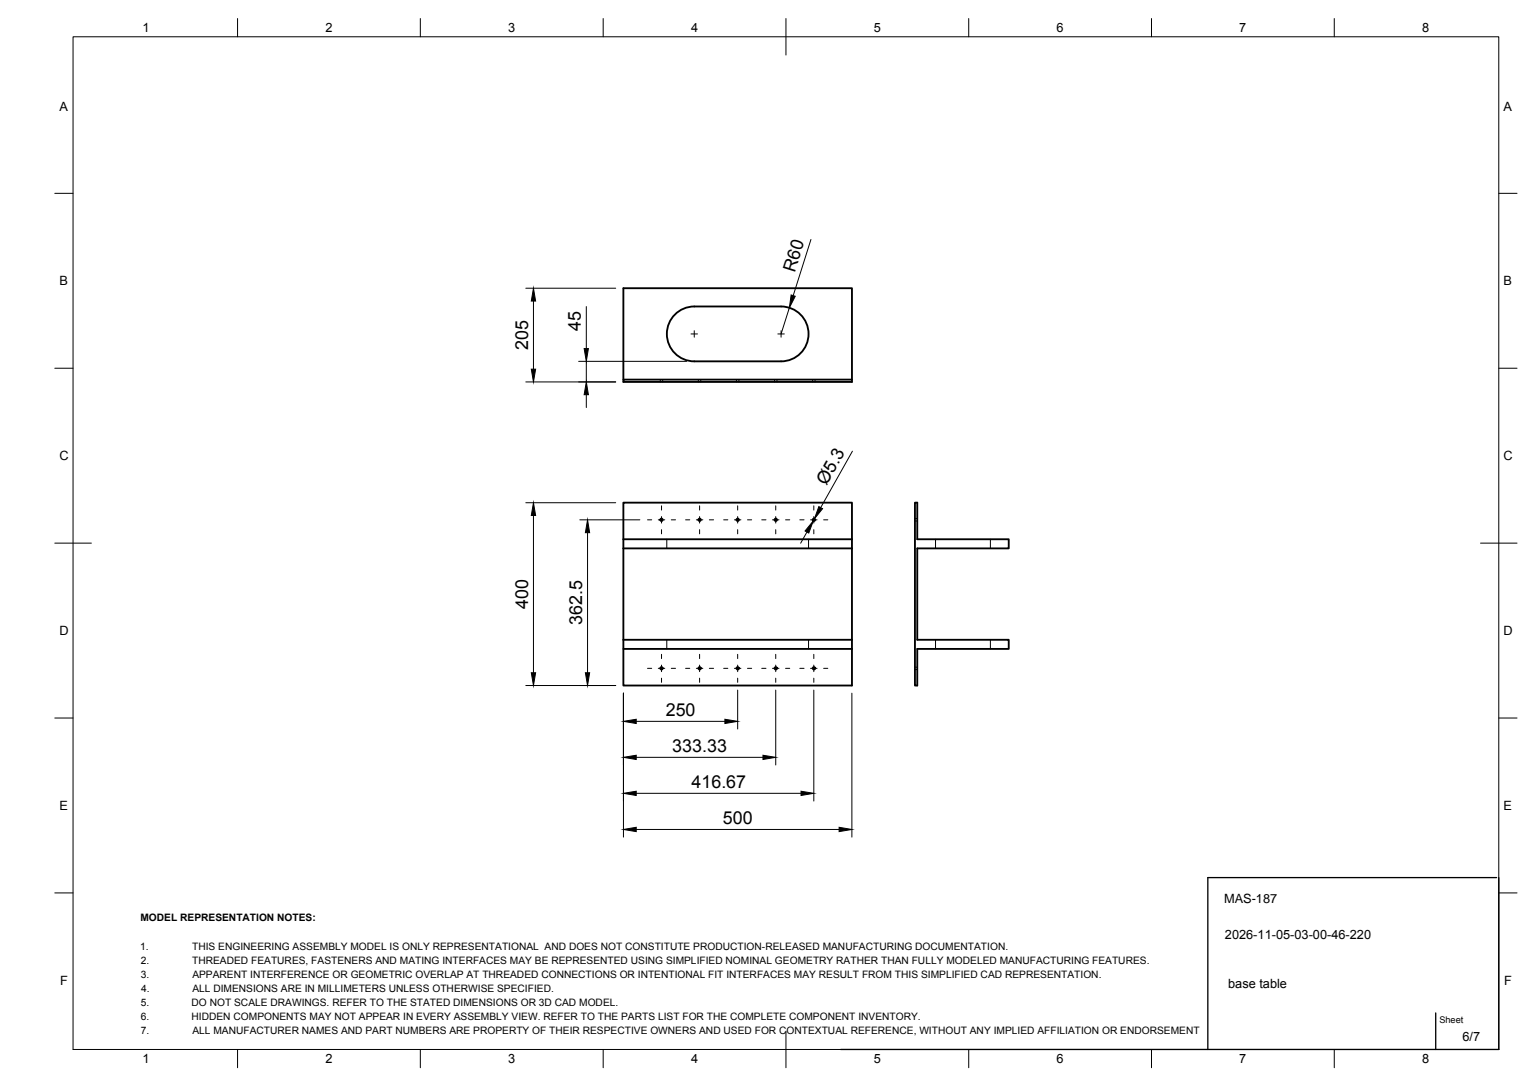
ISO-10303-21;
HEADER;
/* Generated by software containing ST-Developer
 * from STEP Tools, Inc. (www.steptools.com) 
 */

FILE_DESCRIPTION(
/* description */ ('STEP AP214'),
/* implementation_level */ '2;1');

FILE_NAME(
/* name */ 'base table.step',
/* time_stamp */ '2026-11-04T19:00:26-08:00',
/* author */ (''),
/* organization */ (''),
/* preprocessor_version */ 'ST-DEVELOPER v20.2',
/* originating_system */ 'Autodesk Translation Framework v15.17.0.0',
/* authorisation */ '');

FILE_SCHEMA (('AUTOMOTIVE_DESIGN { 1 0 10303 214 3 1 1 }'));
ENDSEC;

DATA;
#10=MECHANICAL_DESIGN_GEOMETRIC_PRESENTATION_REPRESENTATION('',(#271),#5689);
#257=SHAPE_REPRESENTATION_RELATIONSHIP('SRR','None',#5758,#264);
#264=ADVANCED_BREP_SHAPE_REPRESENTATION('',(#278),#5682);
#271=STYLED_ITEM('',(#5802),#278);
#278=MANIFOLD_SOLID_BREP('Body1',#2961);
#285=FACE_BOUND('',#615,.T.);
#286=FACE_BOUND('',#616,.T.);
#287=FACE_BOUND('',#617,.T.);
#288=FACE_BOUND('',#618,.T.);
#289=FACE_BOUND('',#619,.T.);
#290=FACE_BOUND('',#621,.T.);
#291=FACE_BOUND('',#622,.T.);
#292=FACE_BOUND('',#623,.T.);
#293=FACE_BOUND('',#624,.T.);
#294=FACE_BOUND('',#625,.T.);
#295=FACE_BOUND('',#628,.T.);
#296=FACE_BOUND('',#629,.T.);
#297=FACE_BOUND('',#630,.T.);
#298=FACE_BOUND('',#631,.T.);
#299=FACE_BOUND('',#632,.T.);
#300=FACE_BOUND('',#633,.T.);
#301=FACE_BOUND('',#634,.T.);
#302=FACE_BOUND('',#635,.T.);
#303=FACE_BOUND('',#636,.T.);
#304=FACE_BOUND('',#637,.T.);
#305=FACE_BOUND('',#642,.T.);
#306=FACE_BOUND('',#644,.T.);
#307=FACE_BOUND('',#647,.T.);
#308=FACE_BOUND('',#649,.T.);
#343=PLANE('',#3084);
#344=PLANE('',#3085);
#345=PLANE('',#3086);
#346=PLANE('',#3087);
#347=PLANE('',#3088);
#348=PLANE('',#3089);
#349=PLANE('',#3090);
#350=PLANE('',#3091);
#351=PLANE('',#3092);
#352=PLANE('',#3094);
#353=PLANE('',#3096);
#354=PLANE('',#3097);
#355=PLANE('',#3099);
#356=PLANE('',#3101);
#357=PLANE('',#3102);
#358=PLANE('',#3103);
#359=PLANE('',#3106);
#360=PLANE('',#3107);
#442=FACE_OUTER_BOUND('',#601,.T.);
#443=FACE_OUTER_BOUND('',#602,.T.);
#444=FACE_OUTER_BOUND('',#603,.T.);
#445=FACE_OUTER_BOUND('',#604,.T.);
#446=FACE_OUTER_BOUND('',#605,.T.);
#447=FACE_OUTER_BOUND('',#606,.T.);
#448=FACE_OUTER_BOUND('',#607,.T.);
#449=FACE_OUTER_BOUND('',#608,.T.);
#450=FACE_OUTER_BOUND('',#609,.T.);
#451=FACE_OUTER_BOUND('',#610,.T.);
#452=FACE_OUTER_BOUND('',#611,.T.);
#453=FACE_OUTER_BOUND('',#612,.T.);
#454=FACE_OUTER_BOUND('',#613,.T.);
#455=FACE_OUTER_BOUND('',#614,.T.);
#456=FACE_OUTER_BOUND('',#620,.T.);
#457=FACE_OUTER_BOUND('',#626,.T.);
#458=FACE_OUTER_BOUND('',#627,.T.);
#459=FACE_OUTER_BOUND('',#638,.T.);
#460=FACE_OUTER_BOUND('',#639,.T.);
#461=FACE_OUTER_BOUND('',#640,.T.);
#462=FACE_OUTER_BOUND('',#641,.T.);
#463=FACE_OUTER_BOUND('',#643,.T.);
#464=FACE_OUTER_BOUND('',#645,.T.);
#465=FACE_OUTER_BOUND('',#646,.T.);
#466=FACE_OUTER_BOUND('',#648,.T.);
#467=FACE_OUTER_BOUND('',#650,.T.);
#468=FACE_OUTER_BOUND('',#651,.T.);
#469=FACE_OUTER_BOUND('',#652,.T.);
#470=FACE_OUTER_BOUND('',#653,.T.);
#471=FACE_OUTER_BOUND('',#654,.T.);
#472=FACE_OUTER_BOUND('',#655,.T.);
#473=FACE_OUTER_BOUND('',#656,.T.);
#601=EDGE_LOOP('',(#2012,#2013,#2014,#2015));
#602=EDGE_LOOP('',(#2016,#2017,#2018,#2019));
#603=EDGE_LOOP('',(#2020,#2021,#2022,#2023));
#604=EDGE_LOOP('',(#2024,#2025,#2026,#2027));
#605=EDGE_LOOP('',(#2028,#2029,#2030,#2031));
#606=EDGE_LOOP('',(#2032,#2033,#2034,#2035));
#607=EDGE_LOOP('',(#2036,#2037,#2038,#2039));
#608=EDGE_LOOP('',(#2040,#2041,#2042,#2043));
#609=EDGE_LOOP('',(#2044,#2045,#2046,#2047));
#610=EDGE_LOOP('',(#2048,#2049,#2050,#2051));
#611=EDGE_LOOP('',(#2052,#2053,#2054,#2055));
#612=EDGE_LOOP('',(#2056,#2057,#2058,#2059));
#613=EDGE_LOOP('',(#2060,#2061,#2062,#2063));
#614=EDGE_LOOP('',(#2064,#2065,#2066,#2067));
#615=EDGE_LOOP('',(#2068));
#616=EDGE_LOOP('',(#2069));
#617=EDGE_LOOP('',(#2070));
#618=EDGE_LOOP('',(#2071));
#619=EDGE_LOOP('',(#2072));
#620=EDGE_LOOP('',(#2073,#2074,#2075,#2076));
#621=EDGE_LOOP('',(#2077));
#622=EDGE_LOOP('',(#2078));
#623=EDGE_LOOP('',(#2079));
#624=EDGE_LOOP('',(#2080));
#625=EDGE_LOOP('',(#2081));
#626=EDGE_LOOP('',(#2082,#2083,#2084,#2085,#2086,#2087,#2088,#2089,#2090,
#2091,#2092,#2093));
#627=EDGE_LOOP('',(#2094,#2095,#2096,#2097));
#628=EDGE_LOOP('',(#2098));
#629=EDGE_LOOP('',(#2099));
#630=EDGE_LOOP('',(#2100));
#631=EDGE_LOOP('',(#2101));
#632=EDGE_LOOP('',(#2102));
#633=EDGE_LOOP('',(#2103));
#634=EDGE_LOOP('',(#2104));
#635=EDGE_LOOP('',(#2105));
#636=EDGE_LOOP('',(#2106));
#637=EDGE_LOOP('',(#2107));
#638=EDGE_LOOP('',(#2108,#2109,#2110,#2111,#2112,#2113,#2114,#2115,#2116,
#2117,#2118,#2119));
#639=EDGE_LOOP('',(#2120,#2121,#2122,#2123));
#640=EDGE_LOOP('',(#2124,#2125,#2126,#2127));
#641=EDGE_LOOP('',(#2128,#2129,#2130,#2131));
#642=EDGE_LOOP('',(#2132,#2133,#2134,#2135));
#643=EDGE_LOOP('',(#2136,#2137,#2138,#2139));
#644=EDGE_LOOP('',(#2140,#2141,#2142,#2143));
#645=EDGE_LOOP('',(#2144,#2145,#2146,#2147));
#646=EDGE_LOOP('',(#2148,#2149,#2150,#2151));
#647=EDGE_LOOP('',(#2152,#2153,#2154,#2155));
#648=EDGE_LOOP('',(#2156,#2157,#2158,#2159));
#649=EDGE_LOOP('',(#2160,#2161,#2162,#2163));
#650=EDGE_LOOP('',(#2164,#2165,#2166,#2167));
#651=EDGE_LOOP('',(#2168,#2169,#2170,#2171));
#652=EDGE_LOOP('',(#2172,#2173,#2174,#2175));
#653=EDGE_LOOP('',(#2176,#2177,#2178,#2179));
#654=EDGE_LOOP('',(#2180,#2181,#2182,#2183));
#655=EDGE_LOOP('',(#2184,#2185,#2186,#2187));
#656=EDGE_LOOP('',(#2188,#2189,#2190,#2191));
#818=LINE('',#4253,#1049);
#819=LINE('',#4256,#1050);
#820=LINE('',#4262,#1051);
#821=LINE('',#4265,#1052);
#822=LINE('',#4270,#1053);
#823=LINE('',#4276,#1054);
#824=LINE('',#4282,#1055);
#825=LINE('',#4288,#1056);
#826=LINE('',#4294,#1057);
#827=LINE('',#4300,#1058);
#828=LINE('',#4306,#1059);
#829=LINE('',#4312,#1060);
#830=LINE('',#4318,#1061);
#831=LINE('',#4324,#1062);
#832=LINE('',#4329,#1063);
#833=LINE('',#4331,#1064);
#834=LINE('',#4333,#1065);
#835=LINE('',#4334,#1066);
#836=LINE('',#4338,#1067);
#837=LINE('',#4340,#1068);
#838=LINE('',#4342,#1069);
#839=LINE('',#4343,#1070);
#840=LINE('',#4347,#1071);
#841=LINE('',#4349,#1072);
#842=LINE('',#4351,#1073);
#843=LINE('',#4352,#1074);
#844=LINE('',#4355,#1075);
#845=LINE('',#4357,#1076);
#846=LINE('',#4358,#1077);
#847=LINE('',#4360,#1078);
#848=LINE('',#4362,#1079);
#849=LINE('',#4363,#1080);
#850=LINE('',#4365,#1081);
#851=LINE('',#4367,#1082);
#852=LINE('',#4368,#1083);
#853=LINE('',#4371,#1084);
#854=LINE('',#4373,#1085);
#855=LINE('',#4374,#1086);
#856=LINE('',#4376,#1087);
#857=LINE('',#4378,#1088);
#858=LINE('',#4380,#1089);
#859=LINE('',#4381,#1090);
#860=LINE('',#4383,#1091);
#861=LINE('',#4385,#1092);
#862=LINE('',#4386,#1093);
#863=LINE('',#4387,#1094);
#864=LINE('',#4391,#1095);
#865=LINE('',#4393,#1096);
#866=LINE('',#4396,#1097);
#867=LINE('',#4398,#1098);
#868=LINE('',#4402,#1099);
#869=LINE('',#4403,#1100);
#870=LINE('',#4406,#1101);
#871=LINE('',#4408,#1102);
#872=LINE('',#4411,#1103);
#873=LINE('',#4413,#1104);
#874=LINE('',#4417,#1105);
#875=LINE('',#4418,#1106);
#876=LINE('',#4421,#1107);
#877=LINE('',#4423,#1108);
#878=LINE('',#4426,#1109);
#879=LINE('',#4427,#1110);
#1049=VECTOR('',#3377,1000.);
#1050=VECTOR('',#3380,1000.);
#1051=VECTOR('',#3385,1000.);
#1052=VECTOR('',#3388,1000.);
#1053=VECTOR('',#3393,2.64999999999999);
#1054=VECTOR('',#3400,2.64999999999999);
#1055=VECTOR('',#3407,2.64999999999999);
#1056=VECTOR('',#3414,2.64999999999999);
#1057=VECTOR('',#3421,2.64999999999999);
#1058=VECTOR('',#3428,2.64999999999999);
#1059=VECTOR('',#3435,2.64999999999999);
#1060=VECTOR('',#3442,2.64999999999999);
#1061=VECTOR('',#3449,2.64999999999999);
#1062=VECTOR('',#3456,2.64999999999999);
#1063=VECTOR('',#3461,1000.);
#1064=VECTOR('',#3462,1000.);
#1065=VECTOR('',#3463,1000.);
#1066=VECTOR('',#3464,1000.);
#1067=VECTOR('',#3467,1000.);
#1068=VECTOR('',#3468,1000.);
#1069=VECTOR('',#3469,1000.);
#1070=VECTOR('',#3470,1000.);
#1071=VECTOR('',#3473,1000.);
#1072=VECTOR('',#3474,1000.);
#1073=VECTOR('',#3475,1000.);
#1074=VECTOR('',#3476,1000.);
#1075=VECTOR('',#3479,1000.);
#1076=VECTOR('',#3480,1000.);
#1077=VECTOR('',#3481,1000.);
#1078=VECTOR('',#3482,1000.);
#1079=VECTOR('',#3483,1000.);
#1080=VECTOR('',#3484,1000.);
#1081=VECTOR('',#3485,1000.);
#1082=VECTOR('',#3486,1000.);
#1083=VECTOR('',#3487,1000.);
#1084=VECTOR('',#3490,1000.);
#1085=VECTOR('',#3491,1000.);
#1086=VECTOR('',#3492,1000.);
#1087=VECTOR('',#3495,1000.);
#1088=VECTOR('',#3496,1000.);
#1089=VECTOR('',#3497,1000.);
#1090=VECTOR('',#3498,1000.);
#1091=VECTOR('',#3499,1000.);
#1092=VECTOR('',#3500,1000.);
#1093=VECTOR('',#3501,1000.);
#1094=VECTOR('',#3502,1000.);
#1095=VECTOR('',#3509,1000.);
#1096=VECTOR('',#3510,1000.);
#1097=VECTOR('',#3513,1000.);
#1098=VECTOR('',#3516,1000.);
#1099=VECTOR('',#3519,1000.);
#1100=VECTOR('',#3520,1000.);
#1101=VECTOR('',#3525,1000.);
#1102=VECTOR('',#3526,1000.);
#1103=VECTOR('',#3529,1000.);
#1104=VECTOR('',#3532,1000.);
#1105=VECTOR('',#3535,1000.);
#1106=VECTOR('',#3536,1000.);
#1107=VECTOR('',#3541,1000.);
#1108=VECTOR('',#3544,1000.);
#1109=VECTOR('',#3549,1000.);
#1110=VECTOR('',#3550,1000.);
#1280=CIRCLE('',#3049,60.);
#1281=CIRCLE('',#3050,60.);
#1282=CIRCLE('',#3052,60.);
#1283=CIRCLE('',#3053,60.);
#1284=CIRCLE('',#3055,2.64999999999999);
#1285=CIRCLE('',#3056,2.64999999999999);
#1286=CIRCLE('',#3058,2.64999999999999);
#1287=CIRCLE('',#3059,2.64999999999999);
#1288=CIRCLE('',#3061,2.64999999999999);
#1289=CIRCLE('',#3062,2.64999999999999);
#1290=CIRCLE('',#3064,2.64999999999999);
#1291=CIRCLE('',#3065,2.64999999999999);
#1292=CIRCLE('',#3067,2.64999999999999);
#1293=CIRCLE('',#3068,2.64999999999999);
#1294=CIRCLE('',#3070,2.64999999999999);
#1295=CIRCLE('',#3071,2.64999999999999);
#1296=CIRCLE('',#3073,2.64999999999999);
#1297=CIRCLE('',#3074,2.64999999999999);
#1298=CIRCLE('',#3076,2.64999999999999);
#1299=CIRCLE('',#3077,2.64999999999999);
#1300=CIRCLE('',#3079,2.64999999999999);
#1301=CIRCLE('',#3080,2.64999999999999);
#1302=CIRCLE('',#3082,2.64999999999999);
#1303=CIRCLE('',#3083,2.64999999999999);
#1304=CIRCLE('',#3093,60.);
#1305=CIRCLE('',#3095,60.);
#1306=CIRCLE('',#3098,60.);
#1307=CIRCLE('',#3100,60.);
#1395=VERTEX_POINT('',#4249);
#1396=VERTEX_POINT('',#4250);
#1397=VERTEX_POINT('',#4252);
#1398=VERTEX_POINT('',#4254);
#1399=VERTEX_POINT('',#4258);
#1400=VERTEX_POINT('',#4259);
#1401=VERTEX_POINT('',#4261);
#1402=VERTEX_POINT('',#4263);
#1403=VERTEX_POINT('',#4267);
#1404=VERTEX_POINT('',#4269);
#1405=VERTEX_POINT('',#4273);
#1406=VERTEX_POINT('',#4275);
#1407=VERTEX_POINT('',#4279);
#1408=VERTEX_POINT('',#4281);
#1409=VERTEX_POINT('',#4285);
#1410=VERTEX_POINT('',#4287);
#1411=VERTEX_POINT('',#4291);
#1412=VERTEX_POINT('',#4293);
#1413=VERTEX_POINT('',#4297);
#1414=VERTEX_POINT('',#4299);
#1415=VERTEX_POINT('',#4303);
#1416=VERTEX_POINT('',#4305);
#1417=VERTEX_POINT('',#4309);
#1418=VERTEX_POINT('',#4311);
#1419=VERTEX_POINT('',#4315);
#1420=VERTEX_POINT('',#4317);
#1421=VERTEX_POINT('',#4321);
#1422=VERTEX_POINT('',#4323);
#1423=VERTEX_POINT('',#4327);
#1424=VERTEX_POINT('',#4328);
#1425=VERTEX_POINT('',#4330);
#1426=VERTEX_POINT('',#4332);
#1427=VERTEX_POINT('',#4336);
#1428=VERTEX_POINT('',#4337);
#1429=VERTEX_POINT('',#4339);
#1430=VERTEX_POINT('',#4341);
#1431=VERTEX_POINT('',#4345);
#1432=VERTEX_POINT('',#4346);
#1433=VERTEX_POINT('',#4348);
#1434=VERTEX_POINT('',#4350);
#1435=VERTEX_POINT('',#4354);
#1436=VERTEX_POINT('',#4356);
#1437=VERTEX_POINT('',#4359);
#1438=VERTEX_POINT('',#4361);
#1439=VERTEX_POINT('',#4364);
#1440=VERTEX_POINT('',#4366);
#1441=VERTEX_POINT('',#4370);
#1442=VERTEX_POINT('',#4372);
#1443=VERTEX_POINT('',#4377);
#1444=VERTEX_POINT('',#4379);
#1445=VERTEX_POINT('',#4382);
#1446=VERTEX_POINT('',#4384);
#1447=VERTEX_POINT('',#4392);
#1448=VERTEX_POINT('',#4394);
#1449=VERTEX_POINT('',#4399);
#1450=VERTEX_POINT('',#4400);
#1451=VERTEX_POINT('',#4407);
#1452=VERTEX_POINT('',#4409);
#1453=VERTEX_POINT('',#4414);
#1454=VERTEX_POINT('',#4415);
#1634=EDGE_CURVE('',#1395,#1396,#1280,.T.);
#1635=EDGE_CURVE('',#1395,#1397,#818,.T.);
#1636=EDGE_CURVE('',#1397,#1398,#1281,.T.);
#1637=EDGE_CURVE('',#1396,#1398,#819,.T.);
#1638=EDGE_CURVE('',#1399,#1400,#1282,.T.);
#1639=EDGE_CURVE('',#1399,#1401,#820,.T.);
#1640=EDGE_CURVE('',#1401,#1402,#1283,.T.);
#1641=EDGE_CURVE('',#1400,#1402,#821,.T.);
#1642=EDGE_CURVE('',#1403,#1403,#1284,.T.);
#1643=EDGE_CURVE('',#1403,#1404,#822,.T.);
#1644=EDGE_CURVE('',#1404,#1404,#1285,.T.);
#1645=EDGE_CURVE('',#1405,#1405,#1286,.T.);
#1646=EDGE_CURVE('',#1405,#1406,#823,.T.);
#1647=EDGE_CURVE('',#1406,#1406,#1287,.T.);
#1648=EDGE_CURVE('',#1407,#1407,#1288,.T.);
#1649=EDGE_CURVE('',#1407,#1408,#824,.T.);
#1650=EDGE_CURVE('',#1408,#1408,#1289,.T.);
#1651=EDGE_CURVE('',#1409,#1409,#1290,.T.);
#1652=EDGE_CURVE('',#1409,#1410,#825,.T.);
#1653=EDGE_CURVE('',#1410,#1410,#1291,.T.);
#1654=EDGE_CURVE('',#1411,#1411,#1292,.T.);
#1655=EDGE_CURVE('',#1411,#1412,#826,.T.);
#1656=EDGE_CURVE('',#1412,#1412,#1293,.T.);
#1657=EDGE_CURVE('',#1413,#1413,#1294,.T.);
#1658=EDGE_CURVE('',#1413,#1414,#827,.T.);
#1659=EDGE_CURVE('',#1414,#1414,#1295,.T.);
#1660=EDGE_CURVE('',#1415,#1415,#1296,.T.);
#1661=EDGE_CURVE('',#1415,#1416,#828,.T.);
#1662=EDGE_CURVE('',#1416,#1416,#1297,.T.);
#1663=EDGE_CURVE('',#1417,#1417,#1298,.T.);
#1664=EDGE_CURVE('',#1417,#1418,#829,.T.);
#1665=EDGE_CURVE('',#1418,#1418,#1299,.T.);
#1666=EDGE_CURVE('',#1419,#1419,#1300,.T.);
#1667=EDGE_CURVE('',#1419,#1420,#830,.T.);
#1668=EDGE_CURVE('',#1420,#1420,#1301,.T.);
#1669=EDGE_CURVE('',#1421,#1421,#1302,.T.);
#1670=EDGE_CURVE('',#1421,#1422,#831,.T.);
#1671=EDGE_CURVE('',#1422,#1422,#1303,.T.);
#1672=EDGE_CURVE('',#1423,#1424,#832,.T.);
#1673=EDGE_CURVE('',#1423,#1425,#833,.T.);
#1674=EDGE_CURVE('',#1425,#1426,#834,.T.);
#1675=EDGE_CURVE('',#1424,#1426,#835,.T.);
#1676=EDGE_CURVE('',#1427,#1428,#836,.T.);
#1677=EDGE_CURVE('',#1427,#1429,#837,.T.);
#1678=EDGE_CURVE('',#1429,#1430,#838,.T.);
#1679=EDGE_CURVE('',#1428,#1430,#839,.T.);
#1680=EDGE_CURVE('',#1431,#1432,#840,.T.);
#1681=EDGE_CURVE('',#1432,#1433,#841,.T.);
#1682=EDGE_CURVE('',#1434,#1433,#842,.T.);
#1683=EDGE_CURVE('',#1431,#1434,#843,.T.);
#1684=EDGE_CURVE('',#1435,#1430,#844,.T.);
#1685=EDGE_CURVE('',#1436,#1435,#845,.T.);
#1686=EDGE_CURVE('',#1436,#1434,#846,.T.);
#1687=EDGE_CURVE('',#1437,#1433,#847,.T.);
#1688=EDGE_CURVE('',#1437,#1438,#848,.T.);
#1689=EDGE_CURVE('',#1438,#1424,#849,.T.);
#1690=EDGE_CURVE('',#1439,#1426,#850,.T.);
#1691=EDGE_CURVE('',#1439,#1440,#851,.T.);
#1692=EDGE_CURVE('',#1440,#1428,#852,.T.);
#1693=EDGE_CURVE('',#1441,#1435,#853,.T.);
#1694=EDGE_CURVE('',#1442,#1441,#854,.T.);
#1695=EDGE_CURVE('',#1442,#1436,#855,.T.);
#1696=EDGE_CURVE('',#1429,#1441,#856,.T.);
#1697=EDGE_CURVE('',#1443,#1427,#857,.T.);
#1698=EDGE_CURVE('',#1443,#1444,#858,.T.);
#1699=EDGE_CURVE('',#1444,#1425,#859,.T.);
#1700=EDGE_CURVE('',#1445,#1423,#860,.T.);
#1701=EDGE_CURVE('',#1445,#1446,#861,.T.);
#1702=EDGE_CURVE('',#1446,#1432,#862,.T.);
#1703=EDGE_CURVE('',#1431,#1442,#863,.T.);
#1704=EDGE_CURVE('',#1443,#1440,#864,.T.);
#1705=EDGE_CURVE('',#1396,#1447,#865,.T.);
#1706=EDGE_CURVE('',#1447,#1448,#1304,.T.);
#1707=EDGE_CURVE('',#1448,#1395,#866,.T.);
#1708=EDGE_CURVE('',#1444,#1439,#867,.T.);
#1709=EDGE_CURVE('',#1449,#1450,#1305,.T.);
#1710=EDGE_CURVE('',#1398,#1449,#868,.T.);
#1711=EDGE_CURVE('',#1450,#1397,#869,.T.);
#1712=EDGE_CURVE('',#1445,#1438,#870,.T.);
#1713=EDGE_CURVE('',#1400,#1451,#871,.T.);
#1714=EDGE_CURVE('',#1451,#1452,#1306,.T.);
#1715=EDGE_CURVE('',#1452,#1399,#872,.T.);
#1716=EDGE_CURVE('',#1446,#1437,#873,.T.);
#1717=EDGE_CURVE('',#1453,#1454,#1307,.T.);
#1718=EDGE_CURVE('',#1402,#1453,#874,.T.);
#1719=EDGE_CURVE('',#1454,#1401,#875,.T.);
#1720=EDGE_CURVE('',#1452,#1454,#876,.T.);
#1721=EDGE_CURVE('',#1451,#1453,#877,.T.);
#1722=EDGE_CURVE('',#1447,#1449,#878,.T.);
#1723=EDGE_CURVE('',#1448,#1450,#879,.T.);
#2012=ORIENTED_EDGE('',*,*,#1634,.F.);
#2013=ORIENTED_EDGE('',*,*,#1635,.T.);
#2014=ORIENTED_EDGE('',*,*,#1636,.T.);
#2015=ORIENTED_EDGE('',*,*,#1637,.F.);
#2016=ORIENTED_EDGE('',*,*,#1638,.F.);
#2017=ORIENTED_EDGE('',*,*,#1639,.T.);
#2018=ORIENTED_EDGE('',*,*,#1640,.T.);
#2019=ORIENTED_EDGE('',*,*,#1641,.F.);
#2020=ORIENTED_EDGE('',*,*,#1642,.T.);
#2021=ORIENTED_EDGE('',*,*,#1643,.T.);
#2022=ORIENTED_EDGE('',*,*,#1644,.F.);
#2023=ORIENTED_EDGE('',*,*,#1643,.F.);
#2024=ORIENTED_EDGE('',*,*,#1645,.T.);
#2025=ORIENTED_EDGE('',*,*,#1646,.T.);
#2026=ORIENTED_EDGE('',*,*,#1647,.F.);
#2027=ORIENTED_EDGE('',*,*,#1646,.F.);
#2028=ORIENTED_EDGE('',*,*,#1648,.T.);
#2029=ORIENTED_EDGE('',*,*,#1649,.T.);
#2030=ORIENTED_EDGE('',*,*,#1650,.F.);
#2031=ORIENTED_EDGE('',*,*,#1649,.F.);
#2032=ORIENTED_EDGE('',*,*,#1651,.T.);
#2033=ORIENTED_EDGE('',*,*,#1652,.T.);
#2034=ORIENTED_EDGE('',*,*,#1653,.F.);
#2035=ORIENTED_EDGE('',*,*,#1652,.F.);
#2036=ORIENTED_EDGE('',*,*,#1654,.T.);
#2037=ORIENTED_EDGE('',*,*,#1655,.T.);
#2038=ORIENTED_EDGE('',*,*,#1656,.F.);
#2039=ORIENTED_EDGE('',*,*,#1655,.F.);
#2040=ORIENTED_EDGE('',*,*,#1657,.F.);
#2041=ORIENTED_EDGE('',*,*,#1658,.T.);
#2042=ORIENTED_EDGE('',*,*,#1659,.T.);
#2043=ORIENTED_EDGE('',*,*,#1658,.F.);
#2044=ORIENTED_EDGE('',*,*,#1660,.F.);
#2045=ORIENTED_EDGE('',*,*,#1661,.T.);
#2046=ORIENTED_EDGE('',*,*,#1662,.T.);
#2047=ORIENTED_EDGE('',*,*,#1661,.F.);
#2048=ORIENTED_EDGE('',*,*,#1663,.F.);
#2049=ORIENTED_EDGE('',*,*,#1664,.T.);
#2050=ORIENTED_EDGE('',*,*,#1665,.T.);
#2051=ORIENTED_EDGE('',*,*,#1664,.F.);
#2052=ORIENTED_EDGE('',*,*,#1666,.F.);
#2053=ORIENTED_EDGE('',*,*,#1667,.T.);
#2054=ORIENTED_EDGE('',*,*,#1668,.T.);
#2055=ORIENTED_EDGE('',*,*,#1667,.F.);
#2056=ORIENTED_EDGE('',*,*,#1669,.F.);
#2057=ORIENTED_EDGE('',*,*,#1670,.T.);
#2058=ORIENTED_EDGE('',*,*,#1671,.T.);
#2059=ORIENTED_EDGE('',*,*,#1670,.F.);
#2060=ORIENTED_EDGE('',*,*,#1672,.F.);
#2061=ORIENTED_EDGE('',*,*,#1673,.T.);
#2062=ORIENTED_EDGE('',*,*,#1674,.T.);
#2063=ORIENTED_EDGE('',*,*,#1675,.F.);
#2064=ORIENTED_EDGE('',*,*,#1676,.F.);
#2065=ORIENTED_EDGE('',*,*,#1677,.T.);
#2066=ORIENTED_EDGE('',*,*,#1678,.T.);
#2067=ORIENTED_EDGE('',*,*,#1679,.F.);
#2068=ORIENTED_EDGE('',*,*,#1642,.F.);
#2069=ORIENTED_EDGE('',*,*,#1645,.F.);
#2070=ORIENTED_EDGE('',*,*,#1648,.F.);
#2071=ORIENTED_EDGE('',*,*,#1651,.F.);
#2072=ORIENTED_EDGE('',*,*,#1654,.F.);
#2073=ORIENTED_EDGE('',*,*,#1680,.T.);
#2074=ORIENTED_EDGE('',*,*,#1681,.T.);
#2075=ORIENTED_EDGE('',*,*,#1682,.F.);
#2076=ORIENTED_EDGE('',*,*,#1683,.F.);
#2077=ORIENTED_EDGE('',*,*,#1657,.T.);
#2078=ORIENTED_EDGE('',*,*,#1660,.T.);
#2079=ORIENTED_EDGE('',*,*,#1663,.T.);
#2080=ORIENTED_EDGE('',*,*,#1666,.T.);
#2081=ORIENTED_EDGE('',*,*,#1669,.T.);
#2082=ORIENTED_EDGE('',*,*,#1684,.F.);
#2083=ORIENTED_EDGE('',*,*,#1685,.F.);
#2084=ORIENTED_EDGE('',*,*,#1686,.T.);
#2085=ORIENTED_EDGE('',*,*,#1682,.T.);
#2086=ORIENTED_EDGE('',*,*,#1687,.F.);
#2087=ORIENTED_EDGE('',*,*,#1688,.T.);
#2088=ORIENTED_EDGE('',*,*,#1689,.T.);
#2089=ORIENTED_EDGE('',*,*,#1675,.T.);
#2090=ORIENTED_EDGE('',*,*,#1690,.F.);
#2091=ORIENTED_EDGE('',*,*,#1691,.T.);
#2092=ORIENTED_EDGE('',*,*,#1692,.T.);
#2093=ORIENTED_EDGE('',*,*,#1679,.T.);
#2094=ORIENTED_EDGE('',*,*,#1693,.F.);
#2095=ORIENTED_EDGE('',*,*,#1694,.F.);
#2096=ORIENTED_EDGE('',*,*,#1695,.T.);
#2097=ORIENTED_EDGE('',*,*,#1685,.T.);
#2098=ORIENTED_EDGE('',*,*,#1644,.T.);
#2099=ORIENTED_EDGE('',*,*,#1647,.T.);
#2100=ORIENTED_EDGE('',*,*,#1650,.T.);
#2101=ORIENTED_EDGE('',*,*,#1653,.T.);
#2102=ORIENTED_EDGE('',*,*,#1656,.T.);
#2103=ORIENTED_EDGE('',*,*,#1659,.F.);
#2104=ORIENTED_EDGE('',*,*,#1662,.F.);
#2105=ORIENTED_EDGE('',*,*,#1665,.F.);
#2106=ORIENTED_EDGE('',*,*,#1668,.F.);
#2107=ORIENTED_EDGE('',*,*,#1671,.F.);
#2108=ORIENTED_EDGE('',*,*,#1696,.F.);
#2109=ORIENTED_EDGE('',*,*,#1677,.F.);
#2110=ORIENTED_EDGE('',*,*,#1697,.F.);
#2111=ORIENTED_EDGE('',*,*,#1698,.T.);
#2112=ORIENTED_EDGE('',*,*,#1699,.T.);
#2113=ORIENTED_EDGE('',*,*,#1673,.F.);
#2114=ORIENTED_EDGE('',*,*,#1700,.F.);
#2115=ORIENTED_EDGE('',*,*,#1701,.T.);
#2116=ORIENTED_EDGE('',*,*,#1702,.T.);
#2117=ORIENTED_EDGE('',*,*,#1680,.F.);
#2118=ORIENTED_EDGE('',*,*,#1703,.T.);
#2119=ORIENTED_EDGE('',*,*,#1694,.T.);
#2120=ORIENTED_EDGE('',*,*,#1683,.T.);
#2121=ORIENTED_EDGE('',*,*,#1686,.F.);
#2122=ORIENTED_EDGE('',*,*,#1695,.F.);
#2123=ORIENTED_EDGE('',*,*,#1703,.F.);
#2124=ORIENTED_EDGE('',*,*,#1678,.F.);
#2125=ORIENTED_EDGE('',*,*,#1696,.T.);
#2126=ORIENTED_EDGE('',*,*,#1693,.T.);
#2127=ORIENTED_EDGE('',*,*,#1684,.T.);
#2128=ORIENTED_EDGE('',*,*,#1676,.T.);
#2129=ORIENTED_EDGE('',*,*,#1692,.F.);
#2130=ORIENTED_EDGE('',*,*,#1704,.F.);
#2131=ORIENTED_EDGE('',*,*,#1697,.T.);
#2132=ORIENTED_EDGE('',*,*,#1705,.T.);
#2133=ORIENTED_EDGE('',*,*,#1706,.T.);
#2134=ORIENTED_EDGE('',*,*,#1707,.T.);
#2135=ORIENTED_EDGE('',*,*,#1634,.T.);
#2136=ORIENTED_EDGE('',*,*,#1674,.F.);
#2137=ORIENTED_EDGE('',*,*,#1699,.F.);
#2138=ORIENTED_EDGE('',*,*,#1708,.T.);
#2139=ORIENTED_EDGE('',*,*,#1690,.T.);
#2140=ORIENTED_EDGE('',*,*,#1709,.F.);
#2141=ORIENTED_EDGE('',*,*,#1710,.F.);
#2142=ORIENTED_EDGE('',*,*,#1636,.F.);
#2143=ORIENTED_EDGE('',*,*,#1711,.F.);
#2144=ORIENTED_EDGE('',*,*,#1704,.T.);
#2145=ORIENTED_EDGE('',*,*,#1691,.F.);
#2146=ORIENTED_EDGE('',*,*,#1708,.F.);
#2147=ORIENTED_EDGE('',*,*,#1698,.F.);
#2148=ORIENTED_EDGE('',*,*,#1672,.T.);
#2149=ORIENTED_EDGE('',*,*,#1689,.F.);
#2150=ORIENTED_EDGE('',*,*,#1712,.F.);
#2151=ORIENTED_EDGE('',*,*,#1700,.T.);
#2152=ORIENTED_EDGE('',*,*,#1713,.T.);
#2153=ORIENTED_EDGE('',*,*,#1714,.T.);
#2154=ORIENTED_EDGE('',*,*,#1715,.T.);
#2155=ORIENTED_EDGE('',*,*,#1638,.T.);
#2156=ORIENTED_EDGE('',*,*,#1681,.F.);
#2157=ORIENTED_EDGE('',*,*,#1702,.F.);
#2158=ORIENTED_EDGE('',*,*,#1716,.T.);
#2159=ORIENTED_EDGE('',*,*,#1687,.T.);
#2160=ORIENTED_EDGE('',*,*,#1717,.F.);
#2161=ORIENTED_EDGE('',*,*,#1718,.F.);
#2162=ORIENTED_EDGE('',*,*,#1640,.F.);
#2163=ORIENTED_EDGE('',*,*,#1719,.F.);
#2164=ORIENTED_EDGE('',*,*,#1712,.T.);
#2165=ORIENTED_EDGE('',*,*,#1688,.F.);
#2166=ORIENTED_EDGE('',*,*,#1716,.F.);
#2167=ORIENTED_EDGE('',*,*,#1701,.F.);
#2168=ORIENTED_EDGE('',*,*,#1720,.T.);
#2169=ORIENTED_EDGE('',*,*,#1719,.T.);
#2170=ORIENTED_EDGE('',*,*,#1639,.F.);
#2171=ORIENTED_EDGE('',*,*,#1715,.F.);
#2172=ORIENTED_EDGE('',*,*,#1641,.T.);
#2173=ORIENTED_EDGE('',*,*,#1718,.T.);
#2174=ORIENTED_EDGE('',*,*,#1721,.F.);
#2175=ORIENTED_EDGE('',*,*,#1713,.F.);
#2176=ORIENTED_EDGE('',*,*,#1721,.T.);
#2177=ORIENTED_EDGE('',*,*,#1717,.T.);
#2178=ORIENTED_EDGE('',*,*,#1720,.F.);
#2179=ORIENTED_EDGE('',*,*,#1714,.F.);
#2180=ORIENTED_EDGE('',*,*,#1722,.T.);
#2181=ORIENTED_EDGE('',*,*,#1709,.T.);
#2182=ORIENTED_EDGE('',*,*,#1723,.F.);
#2183=ORIENTED_EDGE('',*,*,#1706,.F.);
#2184=ORIENTED_EDGE('',*,*,#1637,.T.);
#2185=ORIENTED_EDGE('',*,*,#1710,.T.);
#2186=ORIENTED_EDGE('',*,*,#1722,.F.);
#2187=ORIENTED_EDGE('',*,*,#1705,.F.);
#2188=ORIENTED_EDGE('',*,*,#1723,.T.);
#2189=ORIENTED_EDGE('',*,*,#1711,.T.);
#2190=ORIENTED_EDGE('',*,*,#1635,.F.);
#2191=ORIENTED_EDGE('',*,*,#1707,.F.);
#2768=CYLINDRICAL_SURFACE('',#3048,60.);
#2769=CYLINDRICAL_SURFACE('',#3051,60.);
#2770=CYLINDRICAL_SURFACE('',#3054,2.64999999999999);
#2771=CYLINDRICAL_SURFACE('',#3057,2.64999999999999);
#2772=CYLINDRICAL_SURFACE('',#3060,2.64999999999999);
#2773=CYLINDRICAL_SURFACE('',#3063,2.64999999999999);
#2774=CYLINDRICAL_SURFACE('',#3066,2.64999999999999);
#2775=CYLINDRICAL_SURFACE('',#3069,2.64999999999999);
#2776=CYLINDRICAL_SURFACE('',#3072,2.64999999999999);
#2777=CYLINDRICAL_SURFACE('',#3075,2.64999999999999);
#2778=CYLINDRICAL_SURFACE('',#3078,2.64999999999999);
#2779=CYLINDRICAL_SURFACE('',#3081,2.64999999999999);
#2780=CYLINDRICAL_SURFACE('',#3104,60.);
#2781=CYLINDRICAL_SURFACE('',#3105,60.);
#2802=ADVANCED_FACE('',(#442),#2768,.F.);
#2803=ADVANCED_FACE('',(#443),#2769,.F.);
#2804=ADVANCED_FACE('',(#444),#2770,.F.);
#2805=ADVANCED_FACE('',(#445),#2771,.F.);
#2806=ADVANCED_FACE('',(#446),#2772,.F.);
#2807=ADVANCED_FACE('',(#447),#2773,.F.);
#2808=ADVANCED_FACE('',(#448),#2774,.F.);
#2809=ADVANCED_FACE('',(#449),#2775,.F.);
#2810=ADVANCED_FACE('',(#450),#2776,.F.);
#2811=ADVANCED_FACE('',(#451),#2777,.F.);
#2812=ADVANCED_FACE('',(#452),#2778,.F.);
#2813=ADVANCED_FACE('',(#453),#2779,.F.);
#2814=ADVANCED_FACE('',(#454),#343,.F.);
#2815=ADVANCED_FACE('',(#455,#285,#286,#287,#288,#289),#344,.F.);
#2816=ADVANCED_FACE('',(#456,#290,#291,#292,#293,#294),#345,.F.);
#2817=ADVANCED_FACE('',(#457),#346,.T.);
#2818=ADVANCED_FACE('',(#458,#295,#296,#297,#298,#299,#300,#301,#302,#303,
#304),#347,.T.);
#2819=ADVANCED_FACE('',(#459),#348,.T.);
#2820=ADVANCED_FACE('',(#460),#349,.F.);
#2821=ADVANCED_FACE('',(#461),#350,.T.);
#2822=ADVANCED_FACE('',(#462,#305),#351,.F.);
#2823=ADVANCED_FACE('',(#463,#306),#352,.T.);
#2824=ADVANCED_FACE('',(#464),#353,.F.);
#2825=ADVANCED_FACE('',(#465,#307),#354,.F.);
#2826=ADVANCED_FACE('',(#466,#308),#355,.T.);
#2827=ADVANCED_FACE('',(#467),#356,.F.);
#2828=ADVANCED_FACE('',(#468),#357,.F.);
#2829=ADVANCED_FACE('',(#469),#358,.F.);
#2830=ADVANCED_FACE('',(#470),#2780,.F.);
#2831=ADVANCED_FACE('',(#471),#2781,.F.);
#2832=ADVANCED_FACE('',(#472),#359,.F.);
#2833=ADVANCED_FACE('',(#473),#360,.F.);
#2961=CLOSED_SHELL('',(#2802,#2803,#2804,#2805,#2806,#2807,#2808,#2809,
#2810,#2811,#2812,#2813,#2814,#2815,#2816,#2817,#2818,#2819,#2820,#2821,
#2822,#2823,#2824,#2825,#2826,#2827,#2828,#2829,#2830,#2831,#2832,#2833));
#3047=AXIS2_PLACEMENT_3D('',#4247,#3371,#3372);
#3048=AXIS2_PLACEMENT_3D('',#4248,#3373,#3374);
#3049=AXIS2_PLACEMENT_3D('',#4251,#3375,#3376);
#3050=AXIS2_PLACEMENT_3D('',#4255,#3378,#3379);
#3051=AXIS2_PLACEMENT_3D('',#4257,#3381,#3382);
#3052=AXIS2_PLACEMENT_3D('',#4260,#3383,#3384);
#3053=AXIS2_PLACEMENT_3D('',#4264,#3386,#3387);
#3054=AXIS2_PLACEMENT_3D('',#4266,#3389,#3390);
#3055=AXIS2_PLACEMENT_3D('',#4268,#3391,#3392);
#3056=AXIS2_PLACEMENT_3D('',#4271,#3394,#3395);
#3057=AXIS2_PLACEMENT_3D('',#4272,#3396,#3397);
#3058=AXIS2_PLACEMENT_3D('',#4274,#3398,#3399);
#3059=AXIS2_PLACEMENT_3D('',#4277,#3401,#3402);
#3060=AXIS2_PLACEMENT_3D('',#4278,#3403,#3404);
#3061=AXIS2_PLACEMENT_3D('',#4280,#3405,#3406);
#3062=AXIS2_PLACEMENT_3D('',#4283,#3408,#3409);
#3063=AXIS2_PLACEMENT_3D('',#4284,#3410,#3411);
#3064=AXIS2_PLACEMENT_3D('',#4286,#3412,#3413);
#3065=AXIS2_PLACEMENT_3D('',#4289,#3415,#3416);
#3066=AXIS2_PLACEMENT_3D('',#4290,#3417,#3418);
#3067=AXIS2_PLACEMENT_3D('',#4292,#3419,#3420);
#3068=AXIS2_PLACEMENT_3D('',#4295,#3422,#3423);
#3069=AXIS2_PLACEMENT_3D('',#4296,#3424,#3425);
#3070=AXIS2_PLACEMENT_3D('',#4298,#3426,#3427);
#3071=AXIS2_PLACEMENT_3D('',#4301,#3429,#3430);
#3072=AXIS2_PLACEMENT_3D('',#4302,#3431,#3432);
#3073=AXIS2_PLACEMENT_3D('',#4304,#3433,#3434);
#3074=AXIS2_PLACEMENT_3D('',#4307,#3436,#3437);
#3075=AXIS2_PLACEMENT_3D('',#4308,#3438,#3439);
#3076=AXIS2_PLACEMENT_3D('',#4310,#3440,#3441);
#3077=AXIS2_PLACEMENT_3D('',#4313,#3443,#3444);
#3078=AXIS2_PLACEMENT_3D('',#4314,#3445,#3446);
#3079=AXIS2_PLACEMENT_3D('',#4316,#3447,#3448);
#3080=AXIS2_PLACEMENT_3D('',#4319,#3450,#3451);
#3081=AXIS2_PLACEMENT_3D('',#4320,#3452,#3453);
#3082=AXIS2_PLACEMENT_3D('',#4322,#3454,#3455);
#3083=AXIS2_PLACEMENT_3D('',#4325,#3457,#3458);
#3084=AXIS2_PLACEMENT_3D('',#4326,#3459,#3460);
#3085=AXIS2_PLACEMENT_3D('',#4335,#3465,#3466);
#3086=AXIS2_PLACEMENT_3D('',#4344,#3471,#3472);
#3087=AXIS2_PLACEMENT_3D('',#4353,#3477,#3478);
#3088=AXIS2_PLACEMENT_3D('',#4369,#3488,#3489);
#3089=AXIS2_PLACEMENT_3D('',#4375,#3493,#3494);
#3090=AXIS2_PLACEMENT_3D('',#4388,#3503,#3504);
#3091=AXIS2_PLACEMENT_3D('',#4389,#3505,#3506);
#3092=AXIS2_PLACEMENT_3D('',#4390,#3507,#3508);
#3093=AXIS2_PLACEMENT_3D('',#4395,#3511,#3512);
#3094=AXIS2_PLACEMENT_3D('',#4397,#3514,#3515);
#3095=AXIS2_PLACEMENT_3D('',#4401,#3517,#3518);
#3096=AXIS2_PLACEMENT_3D('',#4404,#3521,#3522);
#3097=AXIS2_PLACEMENT_3D('',#4405,#3523,#3524);
#3098=AXIS2_PLACEMENT_3D('',#4410,#3527,#3528);
#3099=AXIS2_PLACEMENT_3D('',#4412,#3530,#3531);
#3100=AXIS2_PLACEMENT_3D('',#4416,#3533,#3534);
#3101=AXIS2_PLACEMENT_3D('',#4419,#3537,#3538);
#3102=AXIS2_PLACEMENT_3D('',#4420,#3539,#3540);
#3103=AXIS2_PLACEMENT_3D('',#4422,#3542,#3543);
#3104=AXIS2_PLACEMENT_3D('',#4424,#3545,#3546);
#3105=AXIS2_PLACEMENT_3D('',#4425,#3547,#3548);
#3106=AXIS2_PLACEMENT_3D('',#4428,#3551,#3552);
#3107=AXIS2_PLACEMENT_3D('',#4429,#3553,#3554);
#3371=DIRECTION('axis',(0.,0.,1.));
#3372=DIRECTION('refdir',(1.,0.,0.));
#3373=DIRECTION('center_axis',(0.,0.,1.));
#3374=DIRECTION('ref_axis',(1.,0.,0.));
#3375=DIRECTION('center_axis',(0.,0.,1.));
#3376=DIRECTION('ref_axis',(1.,0.,0.));
#3377=DIRECTION('',(0.,0.,1.));
#3378=DIRECTION('center_axis',(0.,0.,1.));
#3379=DIRECTION('ref_axis',(1.,0.,0.));
#3380=DIRECTION('',(0.,0.,1.));
#3381=DIRECTION('center_axis',(0.,0.,1.));
#3382=DIRECTION('ref_axis',(1.,0.,0.));
#3383=DIRECTION('center_axis',(0.,0.,1.));
#3384=DIRECTION('ref_axis',(1.,0.,0.));
#3385=DIRECTION('',(0.,0.,1.));
#3386=DIRECTION('center_axis',(0.,0.,1.));
#3387=DIRECTION('ref_axis',(1.,0.,0.));
#3388=DIRECTION('',(0.,0.,1.));
#3389=DIRECTION('center_axis',(0.,1.,0.));
#3390=DIRECTION('ref_axis',(0.,0.,-1.));
#3391=DIRECTION('center_axis',(0.,-1.,0.));
#3392=DIRECTION('ref_axis',(0.,0.,-1.));
#3393=DIRECTION('',(0.,1.,0.));
#3394=DIRECTION('center_axis',(0.,-1.,0.));
#3395=DIRECTION('ref_axis',(0.,0.,-1.));
#3396=DIRECTION('center_axis',(0.,1.,0.));
#3397=DIRECTION('ref_axis',(0.,0.,-1.));
#3398=DIRECTION('center_axis',(0.,-1.,0.));
#3399=DIRECTION('ref_axis',(0.,0.,-1.));
#3400=DIRECTION('',(0.,1.,0.));
#3401=DIRECTION('center_axis',(0.,-1.,0.));
#3402=DIRECTION('ref_axis',(0.,0.,-1.));
#3403=DIRECTION('center_axis',(0.,1.,0.));
#3404=DIRECTION('ref_axis',(0.,0.,-1.));
#3405=DIRECTION('center_axis',(0.,-1.,0.));
#3406=DIRECTION('ref_axis',(0.,0.,-1.));
#3407=DIRECTION('',(0.,1.,0.));
#3408=DIRECTION('center_axis',(0.,-1.,0.));
#3409=DIRECTION('ref_axis',(0.,0.,-1.));
#3410=DIRECTION('center_axis',(0.,1.,0.));
#3411=DIRECTION('ref_axis',(0.,0.,-1.));
#3412=DIRECTION('center_axis',(0.,-1.,0.));
#3413=DIRECTION('ref_axis',(0.,0.,-1.));
#3414=DIRECTION('',(0.,1.,0.));
#3415=DIRECTION('center_axis',(0.,-1.,0.));
#3416=DIRECTION('ref_axis',(0.,0.,-1.));
#3417=DIRECTION('center_axis',(0.,1.,0.));
#3418=DIRECTION('ref_axis',(0.,0.,-1.));
#3419=DIRECTION('center_axis',(0.,-1.,0.));
#3420=DIRECTION('ref_axis',(0.,0.,-1.));
#3421=DIRECTION('',(0.,1.,0.));
#3422=DIRECTION('center_axis',(0.,-1.,0.));
#3423=DIRECTION('ref_axis',(0.,0.,-1.));
#3424=DIRECTION('center_axis',(0.,1.,0.));
#3425=DIRECTION('ref_axis',(0.,0.,1.));
#3426=DIRECTION('center_axis',(0.,1.,0.));
#3427=DIRECTION('ref_axis',(0.,0.,1.));
#3428=DIRECTION('',(0.,1.,0.));
#3429=DIRECTION('center_axis',(0.,1.,0.));
#3430=DIRECTION('ref_axis',(0.,0.,1.));
#3431=DIRECTION('center_axis',(0.,1.,0.));
#3432=DIRECTION('ref_axis',(0.,0.,1.));
#3433=DIRECTION('center_axis',(0.,1.,0.));
#3434=DIRECTION('ref_axis',(0.,0.,1.));
#3435=DIRECTION('',(0.,1.,0.));
#3436=DIRECTION('center_axis',(0.,1.,0.));
#3437=DIRECTION('ref_axis',(0.,0.,1.));
#3438=DIRECTION('center_axis',(0.,1.,0.));
#3439=DIRECTION('ref_axis',(0.,0.,1.));
#3440=DIRECTION('center_axis',(0.,1.,0.));
#3441=DIRECTION('ref_axis',(0.,0.,1.));
#3442=DIRECTION('',(0.,1.,0.));
#3443=DIRECTION('center_axis',(0.,1.,0.));
#3444=DIRECTION('ref_axis',(0.,0.,1.));
#3445=DIRECTION('center_axis',(0.,1.,0.));
#3446=DIRECTION('ref_axis',(0.,0.,1.));
#3447=DIRECTION('center_axis',(0.,1.,0.));
#3448=DIRECTION('ref_axis',(0.,0.,1.));
#3449=DIRECTION('',(0.,1.,0.));
#3450=DIRECTION('center_axis',(0.,1.,0.));
#3451=DIRECTION('ref_axis',(0.,0.,1.));
#3452=DIRECTION('center_axis',(0.,1.,0.));
#3453=DIRECTION('ref_axis',(0.,0.,1.));
#3454=DIRECTION('center_axis',(0.,1.,0.));
#3455=DIRECTION('ref_axis',(0.,0.,1.));
#3456=DIRECTION('',(0.,1.,0.));
#3457=DIRECTION('center_axis',(0.,1.,0.));
#3458=DIRECTION('ref_axis',(0.,0.,1.));
#3459=DIRECTION('center_axis',(0.,1.,0.));
#3460=DIRECTION('ref_axis',(0.,0.,1.));
#3461=DIRECTION('',(1.,0.,0.));
#3462=DIRECTION('',(0.,0.,-1.));
#3463=DIRECTION('',(1.,0.,0.));
#3464=DIRECTION('',(0.,0.,-1.));
#3465=DIRECTION('center_axis',(0.,1.,0.));
#3466=DIRECTION('ref_axis',(0.,0.,1.));
#3467=DIRECTION('',(1.,0.,0.));
#3468=DIRECTION('',(0.,0.,-1.));
#3469=DIRECTION('',(1.,0.,0.));
#3470=DIRECTION('',(0.,0.,-1.));
#3471=DIRECTION('center_axis',(0.,1.,0.));
#3472=DIRECTION('ref_axis',(0.,0.,1.));
#3473=DIRECTION('',(0.,0.,-1.));
#3474=DIRECTION('',(1.,0.,0.));
#3475=DIRECTION('',(0.,0.,-1.));
#3476=DIRECTION('',(1.,0.,0.));
#3477=DIRECTION('center_axis',(1.,0.,0.));
#3478=DIRECTION('ref_axis',(0.,0.,-1.));
#3479=DIRECTION('',(0.,-1.,0.));
#3480=DIRECTION('',(0.,0.,-1.));
#3481=DIRECTION('',(0.,-1.,0.));
#3482=DIRECTION('',(0.,1.,0.));
#3483=DIRECTION('',(0.,0.,-1.));
#3484=DIRECTION('',(0.,1.,0.));
#3485=DIRECTION('',(0.,1.,0.));
#3486=DIRECTION('',(0.,0.,-1.));
#3487=DIRECTION('',(0.,1.,0.));
#3488=DIRECTION('center_axis',(0.,1.,0.));
#3489=DIRECTION('ref_axis',(0.,0.,1.));
#3490=DIRECTION('',(1.,0.,0.));
#3491=DIRECTION('',(0.,0.,-1.));
#3492=DIRECTION('',(1.,0.,0.));
#3493=DIRECTION('center_axis',(-1.,0.,0.));
#3494=DIRECTION('ref_axis',(0.,0.,1.));
#3495=DIRECTION('',(0.,1.,0.));
#3496=DIRECTION('',(0.,1.,0.));
#3497=DIRECTION('',(0.,0.,1.));
#3498=DIRECTION('',(0.,1.,0.));
#3499=DIRECTION('',(0.,1.,0.));
#3500=DIRECTION('',(0.,0.,1.));
#3501=DIRECTION('',(0.,1.,0.));
#3502=DIRECTION('',(0.,1.,0.));
#3503=DIRECTION('center_axis',(0.,0.,-1.));
#3504=DIRECTION('ref_axis',(-1.,0.,0.));
#3505=DIRECTION('center_axis',(0.,0.,-1.));
#3506=DIRECTION('ref_axis',(-1.,0.,0.));
#3507=DIRECTION('center_axis',(0.,0.,1.));
#3508=DIRECTION('ref_axis',(1.,0.,0.));
#3509=DIRECTION('',(1.,0.,0.));
#3510=DIRECTION('',(-1.,-2.19122965386544E-16,0.));
#3511=DIRECTION('center_axis',(0.,0.,1.));
#3512=DIRECTION('ref_axis',(1.,0.,0.));
#3513=DIRECTION('',(1.,1.46081976924363E-16,0.));
#3514=DIRECTION('center_axis',(0.,0.,1.));
#3515=DIRECTION('ref_axis',(1.,0.,0.));
#3516=DIRECTION('',(1.,0.,0.));
#3517=DIRECTION('center_axis',(0.,0.,1.));
#3518=DIRECTION('ref_axis',(1.,0.,0.));
#3519=DIRECTION('',(-1.,-2.19122965386544E-16,0.));
#3520=DIRECTION('',(1.,1.46081976924363E-16,0.));
#3521=DIRECTION('center_axis',(0.,1.,0.));
#3522=DIRECTION('ref_axis',(-1.,0.,0.));
#3523=DIRECTION('center_axis',(0.,0.,1.));
#3524=DIRECTION('ref_axis',(1.,0.,0.));
#3525=DIRECTION('',(1.,0.,0.));
#3526=DIRECTION('',(-1.,-2.19122965386544E-16,0.));
#3527=DIRECTION('center_axis',(0.,0.,1.));
#3528=DIRECTION('ref_axis',(1.,0.,0.));
#3529=DIRECTION('',(1.,1.46081976924363E-16,0.));
#3530=DIRECTION('center_axis',(0.,0.,1.));
#3531=DIRECTION('ref_axis',(1.,0.,0.));
#3532=DIRECTION('',(1.,0.,0.));
#3533=DIRECTION('center_axis',(0.,0.,1.));
#3534=DIRECTION('ref_axis',(1.,0.,0.));
#3535=DIRECTION('',(-1.,-2.19122965386544E-16,0.));
#3536=DIRECTION('',(1.,1.46081976924363E-16,0.));
#3537=DIRECTION('center_axis',(0.,1.,0.));
#3538=DIRECTION('ref_axis',(-1.,0.,0.));
#3539=DIRECTION('center_axis',(1.46081976924363E-16,-1.,0.));
#3540=DIRECTION('ref_axis',(1.,1.46081976924363E-16,0.));
#3541=DIRECTION('',(0.,0.,1.));
#3542=DIRECTION('center_axis',(-2.19122965386544E-16,1.,0.));
#3543=DIRECTION('ref_axis',(-1.,-2.19122965386544E-16,0.));
#3544=DIRECTION('',(0.,0.,1.));
#3545=DIRECTION('center_axis',(0.,0.,1.));
#3546=DIRECTION('ref_axis',(-1.,1.22464679914735E-16,0.));
#3547=DIRECTION('center_axis',(0.,0.,1.));
#3548=DIRECTION('ref_axis',(-1.,1.22464679914735E-16,0.));
#3549=DIRECTION('',(0.,0.,1.));
#3550=DIRECTION('',(0.,0.,1.));
#3551=DIRECTION('center_axis',(-2.19122965386544E-16,1.,0.));
#3552=DIRECTION('ref_axis',(-1.,-2.19122965386544E-16,0.));
#3553=DIRECTION('center_axis',(1.46081976924363E-16,-1.,0.));
#3554=DIRECTION('ref_axis',(1.,1.46081976924363E-16,0.));
#4247=CARTESIAN_POINT('',(0.,0.,0.));
#4248=CARTESIAN_POINT('Origin',(315.,-130.,-200.));
#4249=CARTESIAN_POINT('',(315.,-190.,-120.));
#4250=CARTESIAN_POINT('',(315.,-70.,-120.));
#4251=CARTESIAN_POINT('Origin',(315.,-130.,-120.));
#4252=CARTESIAN_POINT('',(315.,-190.,-100.));
#4253=CARTESIAN_POINT('',(315.,-190.,-200.));
#4254=CARTESIAN_POINT('',(315.,-70.,-100.));
#4255=CARTESIAN_POINT('Origin',(315.,-130.,-100.));
#4256=CARTESIAN_POINT('',(315.,-70.,-200.));
#4257=CARTESIAN_POINT('Origin',(315.,-130.,-200.));
#4258=CARTESIAN_POINT('',(315.,-190.,100.));
#4259=CARTESIAN_POINT('',(315.,-70.,100.));
#4260=CARTESIAN_POINT('Origin',(315.,-130.,100.));
#4261=CARTESIAN_POINT('',(315.,-190.,120.));
#4262=CARTESIAN_POINT('',(315.,-190.,-200.));
#4263=CARTESIAN_POINT('',(315.,-70.,120.));
#4264=CARTESIAN_POINT('Origin',(315.,-130.,120.));
#4265=CARTESIAN_POINT('',(315.,-70.,-200.));
#4266=CARTESIAN_POINT('Origin',(136.666666666667,-25.,-162.5));
#4267=CARTESIAN_POINT('',(136.666666666667,-30.,-159.85));
#4268=CARTESIAN_POINT('Origin',(136.666666666667,-30.,-162.5));
#4269=CARTESIAN_POINT('',(136.666666666667,-25.,-159.85));
#4270=CARTESIAN_POINT('',(136.666666666667,-25.,-159.85));
#4271=CARTESIAN_POINT('Origin',(136.666666666667,-25.,-162.5));
#4272=CARTESIAN_POINT('Origin',(220.,-25.,-162.5));
#4273=CARTESIAN_POINT('',(220.,-30.,-159.85));
#4274=CARTESIAN_POINT('Origin',(220.,-30.,-162.5));
#4275=CARTESIAN_POINT('',(220.,-25.,-159.85));
#4276=CARTESIAN_POINT('',(220.,-25.,-159.85));
#4277=CARTESIAN_POINT('Origin',(220.,-25.,-162.5));
#4278=CARTESIAN_POINT('Origin',(303.333333333333,-25.,-162.5));
#4279=CARTESIAN_POINT('',(303.333333333333,-30.,-159.85));
#4280=CARTESIAN_POINT('Origin',(303.333333333333,-30.,-162.5));
#4281=CARTESIAN_POINT('',(303.333333333333,-25.,-159.85));
#4282=CARTESIAN_POINT('',(303.333333333333,-25.,-159.85));
#4283=CARTESIAN_POINT('Origin',(303.333333333333,-25.,-162.5));
#4284=CARTESIAN_POINT('Origin',(386.666666666667,-25.,-162.5));
#4285=CARTESIAN_POINT('',(386.666666666667,-30.,-159.85));
#4286=CARTESIAN_POINT('Origin',(386.666666666667,-30.,-162.5));
#4287=CARTESIAN_POINT('',(386.666666666667,-25.,-159.85));
#4288=CARTESIAN_POINT('',(386.666666666667,-25.,-159.85));
#4289=CARTESIAN_POINT('Origin',(386.666666666667,-25.,-162.5));
#4290=CARTESIAN_POINT('Origin',(53.3333333333333,-25.,-162.5));
#4291=CARTESIAN_POINT('',(53.3333333333333,-30.,-159.85));
#4292=CARTESIAN_POINT('Origin',(53.3333333333333,-30.,-162.5));
#4293=CARTESIAN_POINT('',(53.3333333333333,-25.,-159.85));
#4294=CARTESIAN_POINT('',(53.3333333333333,-25.,-159.85));
#4295=CARTESIAN_POINT('Origin',(53.3333333333333,-25.,-162.5));
#4296=CARTESIAN_POINT('Origin',(53.3333333333333,-25.,162.5));
#4297=CARTESIAN_POINT('',(53.3333333333333,-30.,159.85));
#4298=CARTESIAN_POINT('Origin',(53.3333333333333,-30.,162.5));
#4299=CARTESIAN_POINT('',(53.3333333333333,-25.,159.85));
#4300=CARTESIAN_POINT('',(53.3333333333333,-25.,159.85));
#4301=CARTESIAN_POINT('Origin',(53.3333333333333,-25.,162.5));
#4302=CARTESIAN_POINT('Origin',(136.666666666667,-25.,162.5));
#4303=CARTESIAN_POINT('',(136.666666666667,-30.,159.85));
#4304=CARTESIAN_POINT('Origin',(136.666666666667,-30.,162.5));
#4305=CARTESIAN_POINT('',(136.666666666667,-25.,159.85));
#4306=CARTESIAN_POINT('',(136.666666666667,-25.,159.85));
#4307=CARTESIAN_POINT('Origin',(136.666666666667,-25.,162.5));
#4308=CARTESIAN_POINT('Origin',(220.,-25.,162.5));
#4309=CARTESIAN_POINT('',(220.,-30.,159.85));
#4310=CARTESIAN_POINT('Origin',(220.,-30.,162.5));
#4311=CARTESIAN_POINT('',(220.,-25.,159.85));
#4312=CARTESIAN_POINT('',(220.,-25.,159.85));
#4313=CARTESIAN_POINT('Origin',(220.,-25.,162.5));
#4314=CARTESIAN_POINT('Origin',(303.333333333333,-25.,162.5));
#4315=CARTESIAN_POINT('',(303.333333333333,-30.,159.85));
#4316=CARTESIAN_POINT('Origin',(303.333333333333,-30.,162.5));
#4317=CARTESIAN_POINT('',(303.333333333333,-25.,159.85));
#4318=CARTESIAN_POINT('',(303.333333333333,-25.,159.85));
#4319=CARTESIAN_POINT('Origin',(303.333333333333,-25.,162.5));
#4320=CARTESIAN_POINT('Origin',(386.666666666667,-25.,162.5));
#4321=CARTESIAN_POINT('',(386.666666666667,-30.,159.85));
#4322=CARTESIAN_POINT('Origin',(386.666666666667,-30.,162.5));
#4323=CARTESIAN_POINT('',(386.666666666667,-25.,159.85));
#4324=CARTESIAN_POINT('',(386.666666666667,-25.,159.85));
#4325=CARTESIAN_POINT('Origin',(386.666666666667,-25.,162.5));
#4326=CARTESIAN_POINT('Origin',(-30.,-30.,200.));
#4327=CARTESIAN_POINT('',(-30.,-30.,100.));
#4328=CARTESIAN_POINT('',(470.,-30.,100.));
#4329=CARTESIAN_POINT('',(-30.,-30.,100.));
#4330=CARTESIAN_POINT('',(-30.,-30.,-100.));
#4331=CARTESIAN_POINT('',(-30.,-30.,200.));
#4332=CARTESIAN_POINT('',(470.,-30.,-100.));
#4333=CARTESIAN_POINT('',(-30.,-30.,-100.));
#4334=CARTESIAN_POINT('',(470.,-30.,200.));
#4335=CARTESIAN_POINT('Origin',(-30.,-30.,200.));
#4336=CARTESIAN_POINT('',(-30.,-30.,-120.));
#4337=CARTESIAN_POINT('',(470.,-30.,-120.));
#4338=CARTESIAN_POINT('',(-30.,-30.,-120.));
#4339=CARTESIAN_POINT('',(-30.,-30.,-200.));
#4340=CARTESIAN_POINT('',(-30.,-30.,200.));
#4341=CARTESIAN_POINT('',(470.,-30.,-200.));
#4342=CARTESIAN_POINT('',(-30.,-30.,-200.));
#4343=CARTESIAN_POINT('',(470.,-30.,200.));
#4344=CARTESIAN_POINT('Origin',(-30.,-30.,200.));
#4345=CARTESIAN_POINT('',(-30.,-30.,200.));
#4346=CARTESIAN_POINT('',(-30.,-30.,120.));
#4347=CARTESIAN_POINT('',(-30.,-30.,200.));
#4348=CARTESIAN_POINT('',(470.,-30.,120.));
#4349=CARTESIAN_POINT('',(-30.,-30.,120.));
#4350=CARTESIAN_POINT('',(470.,-30.,200.));
#4351=CARTESIAN_POINT('',(470.,-30.,200.));
#4352=CARTESIAN_POINT('',(-30.,-30.,200.));
#4353=CARTESIAN_POINT('Origin',(470.,-25.,200.));
#4354=CARTESIAN_POINT('',(470.,-25.,-200.));
#4355=CARTESIAN_POINT('',(470.,-25.,-200.));
#4356=CARTESIAN_POINT('',(470.,-25.,200.));
#4357=CARTESIAN_POINT('',(470.,-25.,200.));
#4358=CARTESIAN_POINT('',(470.,-25.,200.));
#4359=CARTESIAN_POINT('',(470.,-230.,120.));
#4360=CARTESIAN_POINT('',(470.,-230.,120.));
#4361=CARTESIAN_POINT('',(470.,-230.,100.));
#4362=CARTESIAN_POINT('',(470.,-230.,120.));
#4363=CARTESIAN_POINT('',(470.,-230.,100.));
#4364=CARTESIAN_POINT('',(470.,-230.,-100.));
#4365=CARTESIAN_POINT('',(470.,-230.,-100.));
#4366=CARTESIAN_POINT('',(470.,-230.,-120.));
#4367=CARTESIAN_POINT('',(470.,-230.,-100.));
#4368=CARTESIAN_POINT('',(470.,-230.,-120.));
#4369=CARTESIAN_POINT('Origin',(-30.,-25.,200.));
#4370=CARTESIAN_POINT('',(-30.,-25.,-200.));
#4371=CARTESIAN_POINT('',(-30.,-25.,-200.));
#4372=CARTESIAN_POINT('',(-30.,-25.,200.));
#4373=CARTESIAN_POINT('',(-30.,-25.,200.));
#4374=CARTESIAN_POINT('',(-30.,-25.,200.));
#4375=CARTESIAN_POINT('Origin',(-30.,-30.,200.));
#4376=CARTESIAN_POINT('',(-30.,-30.,-200.));
#4377=CARTESIAN_POINT('',(-30.,-230.,-120.));
#4378=CARTESIAN_POINT('',(-30.,-230.,-120.));
#4379=CARTESIAN_POINT('',(-30.,-230.,-100.));
#4380=CARTESIAN_POINT('',(-30.,-230.,-120.));
#4381=CARTESIAN_POINT('',(-30.,-230.,-100.));
#4382=CARTESIAN_POINT('',(-30.,-230.,100.));
#4383=CARTESIAN_POINT('',(-30.,-230.,100.));
#4384=CARTESIAN_POINT('',(-30.,-230.,120.));
#4385=CARTESIAN_POINT('',(-30.,-230.,100.));
#4386=CARTESIAN_POINT('',(-30.,-230.,120.));
#4387=CARTESIAN_POINT('',(-30.,-30.,200.));
#4388=CARTESIAN_POINT('Origin',(0.,0.,200.));
#4389=CARTESIAN_POINT('Origin',(0.,0.,-200.));
#4390=CARTESIAN_POINT('Origin',(-30.,-230.,-120.));
#4391=CARTESIAN_POINT('',(-30.,-230.,-120.));
#4392=CARTESIAN_POINT('',(125.,-70.0000000000001,-120.));
#4393=CARTESIAN_POINT('',(-30.0000000000001,-70.0000000000001,-120.));
#4394=CARTESIAN_POINT('',(125.,-190.,-120.));
#4395=CARTESIAN_POINT('Origin',(125.,-130.,-120.));
#4396=CARTESIAN_POINT('',(-30.,-190.,-120.));
#4397=CARTESIAN_POINT('Origin',(-30.,-230.,-100.));
#4398=CARTESIAN_POINT('',(-30.,-230.,-100.));
#4399=CARTESIAN_POINT('',(125.,-70.0000000000001,-100.));
#4400=CARTESIAN_POINT('',(125.,-190.,-100.));
#4401=CARTESIAN_POINT('Origin',(125.,-130.,-100.));
#4402=CARTESIAN_POINT('',(-30.0000000000001,-70.0000000000001,-100.));
#4403=CARTESIAN_POINT('',(-30.,-190.,-100.));
#4404=CARTESIAN_POINT('Origin',(0.,-230.,0.));
#4405=CARTESIAN_POINT('Origin',(-30.,-230.,100.));
#4406=CARTESIAN_POINT('',(-30.,-230.,100.));
#4407=CARTESIAN_POINT('',(125.,-70.0000000000001,100.));
#4408=CARTESIAN_POINT('',(-30.0000000000001,-70.0000000000001,100.));
#4409=CARTESIAN_POINT('',(125.,-190.,100.));
#4410=CARTESIAN_POINT('Origin',(125.,-130.,100.));
#4411=CARTESIAN_POINT('',(-30.,-190.,100.));
#4412=CARTESIAN_POINT('Origin',(-30.,-230.,120.));
#4413=CARTESIAN_POINT('',(-30.,-230.,120.));
#4414=CARTESIAN_POINT('',(125.,-70.0000000000001,120.));
#4415=CARTESIAN_POINT('',(125.,-190.,120.));
#4416=CARTESIAN_POINT('Origin',(125.,-130.,120.));
#4417=CARTESIAN_POINT('',(-30.0000000000001,-70.0000000000001,120.));
#4418=CARTESIAN_POINT('',(-30.,-190.,120.));
#4419=CARTESIAN_POINT('Origin',(0.,-230.,0.));
#4420=CARTESIAN_POINT('Origin',(125.,-190.,-200.));
#4421=CARTESIAN_POINT('',(125.,-190.,-200.));
#4422=CARTESIAN_POINT('Origin',(125.,-70.0000000000001,-200.));
#4423=CARTESIAN_POINT('',(125.,-70.0000000000001,-200.));
#4424=CARTESIAN_POINT('Origin',(125.,-130.,-200.));
#4425=CARTESIAN_POINT('Origin',(125.,-130.,-200.));
#4426=CARTESIAN_POINT('',(125.,-70.0000000000001,-200.));
#4427=CARTESIAN_POINT('',(125.,-190.,-200.));
#4428=CARTESIAN_POINT('Origin',(125.,-70.0000000000001,-200.));
#4429=CARTESIAN_POINT('Origin',(125.,-190.,-200.));
#5673=UNCERTAINTY_MEASURE_WITH_UNIT(LENGTH_MEASURE(0.01),#5690,
'DISTANCE_ACCURACY_VALUE',
'Maximum model space distance between geometric entities at asserted c
onnectivities');
#5680=UNCERTAINTY_MEASURE_WITH_UNIT(LENGTH_MEASURE(0.01),#5690,
'DISTANCE_ACCURACY_VALUE',
'Maximum model space distance between geometric entities at asserted c
onnectivities');
#5682=(
GEOMETRIC_REPRESENTATION_CONTEXT(3)
GLOBAL_UNCERTAINTY_ASSIGNED_CONTEXT((#5673))
GLOBAL_UNIT_ASSIGNED_CONTEXT((#5690,#5692,#5693))
REPRESENTATION_CONTEXT('','3D')
);
#5689=(
GEOMETRIC_REPRESENTATION_CONTEXT(3)
GLOBAL_UNCERTAINTY_ASSIGNED_CONTEXT((#5680))
GLOBAL_UNIT_ASSIGNED_CONTEXT((#5690,#5692,#5693))
REPRESENTATION_CONTEXT('','3D')
);
#5690=(
LENGTH_UNIT()
NAMED_UNIT(*)
SI_UNIT(.MILLI.,.METRE.)
);
#5692=(
NAMED_UNIT(*)
PLANE_ANGLE_UNIT()
SI_UNIT($,.RADIAN.)
);
#5693=(
NAMED_UNIT(*)
SI_UNIT($,.STERADIAN.)
SOLID_ANGLE_UNIT()
);
#5695=SHAPE_DEFINITION_REPRESENTATION(#5703,#5758);
#5703=PRODUCT_DEFINITION_SHAPE('',$,#5767);
#5758=SHAPE_REPRESENTATION('',(#3047),#5682);
#5765=PRODUCT_DEFINITION_CONTEXT('part definition',#5791,'design');
#5767=PRODUCT_DEFINITION('base table','base table',#5775,#5765);
#5775=PRODUCT_DEFINITION_FORMATION('',$,#5794);
#5791=APPLICATION_CONTEXT(
'Core Data for Automotive Mechanical Design Process');
#5792=PRODUCT_CONTEXT('part definition',#5791,'mechanical');
#5794=PRODUCT('base table','base table',$,(#5792));
#5802=PRESENTATION_STYLE_ASSIGNMENT((#5808));
#5808=SURFACE_STYLE_USAGE(.BOTH.,#5814);
#5814=SURFACE_SIDE_STYLE('',(#5820));
#5820=SURFACE_STYLE_FILL_AREA(#5826);
#5826=FILL_AREA_STYLE('Opaque(20,51,87)',(#5832));
#5832=FILL_AREA_STYLE_COLOUR('Opaque(20,51,87)',#5838);
#5838=COLOUR_RGB('Opaque(20,51,87)',0.0784313725490196,0.2,0.341176470588235);
ENDSEC;
END-ISO-10303-21;
